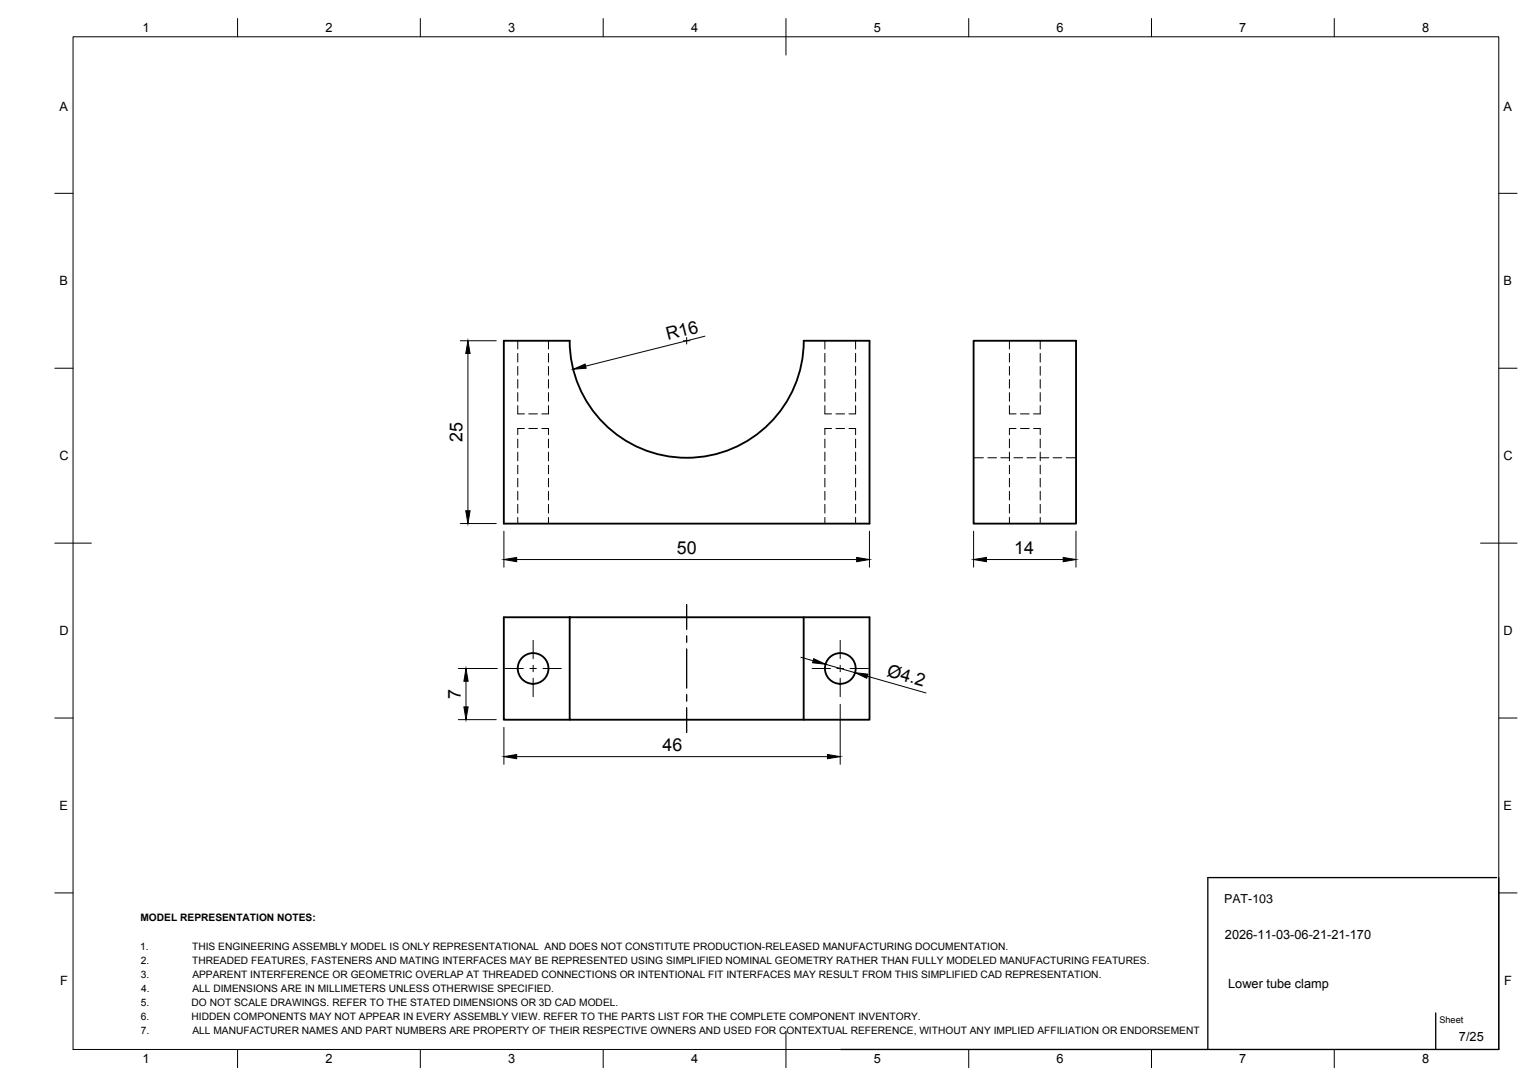
ISO-10303-21;
HEADER;
/* Generated by software containing ST-Developer
 * from STEP Tools, Inc. (www.steptools.com) 
 */

FILE_DESCRIPTION(
/* description */ ('Telescoping shaft support with lock collar'),
/* implementation_level */ '2;1');

FILE_NAME(
/* name */ 'Lower tube clamp.step',
/* time_stamp */ '2026-10-27T10:48:51-07:00',
/* author */ (''),
/* organization */ (''),
/* preprocessor_version */ 'ST-DEVELOPER v20.2',
/* originating_system */ 'Autodesk Translation Framework v15.17.0.0',
/* authorisation */ '');

FILE_SCHEMA (('AUTOMOTIVE_DESIGN { 1 0 10303 214 3 1 1 }'));
ENDSEC;

DATA;
#10=MECHANICAL_DESIGN_GEOMETRIC_PRESENTATION_REPRESENTATION('',(#243),#7349);
#203=SHAPE_REPRESENTATION_RELATIONSHIP('SRR','None',#7445,#223);
#223=ADVANCED_BREP_SHAPE_REPRESENTATION('',(#263),#7329);
#243=STYLED_ITEM('',(#7613),#263);
#263=MANIFOLD_SOLID_BREP('Body1',#3966);
#297=FACE_BOUND('',#780,.T.);
#298=FACE_BOUND('',#785,.T.);
#299=FACE_BOUND('',#787,.T.);
#300=FACE_BOUND('',#788,.T.);
#375=PLANE('',#4297);
#376=PLANE('',#4301);
#377=PLANE('',#4305);
#378=PLANE('',#4309);
#379=PLANE('',#4313);
#380=PLANE('',#4314);
#381=PLANE('',#4315);
#382=PLANE('',#4316);
#383=PLANE('',#4317);
#384=PLANE('',#4318);
#385=PLANE('',#4319);
#525=FACE_OUTER_BOUND('',#769,.T.);
#526=FACE_OUTER_BOUND('',#770,.T.);
#527=FACE_OUTER_BOUND('',#771,.T.);
#528=FACE_OUTER_BOUND('',#772,.T.);
#529=FACE_OUTER_BOUND('',#773,.T.);
#530=FACE_OUTER_BOUND('',#774,.T.);
#531=FACE_OUTER_BOUND('',#775,.T.);
#532=FACE_OUTER_BOUND('',#776,.T.);
#533=FACE_OUTER_BOUND('',#777,.T.);
#534=FACE_OUTER_BOUND('',#778,.T.);
#535=FACE_OUTER_BOUND('',#779,.T.);
#536=FACE_OUTER_BOUND('',#781,.T.);
#537=FACE_OUTER_BOUND('',#782,.T.);
#538=FACE_OUTER_BOUND('',#783,.T.);
#539=FACE_OUTER_BOUND('',#784,.T.);
#540=FACE_OUTER_BOUND('',#786,.T.);
#769=EDGE_LOOP('',(#2822,#2823,#2824,#2825));
#770=EDGE_LOOP('',(#2826));
#771=EDGE_LOOP('',(#2827,#2828,#2829,#2830));
#772=EDGE_LOOP('',(#2831));
#773=EDGE_LOOP('',(#2832,#2833,#2834,#2835));
#774=EDGE_LOOP('',(#2836));
#775=EDGE_LOOP('',(#2837,#2838,#2839,#2840));
#776=EDGE_LOOP('',(#2841));
#777=EDGE_LOOP('',(#2842,#2843,#2844,#2845));
#778=EDGE_LOOP('',(#2846,#2847,#2848,#2849,#2850,#2851));
#779=EDGE_LOOP('',(#2852,#2853,#2854,#2855));
#780=EDGE_LOOP('',(#2856));
#781=EDGE_LOOP('',(#2857,#2858,#2859,#2860));
#782=EDGE_LOOP('',(#2861,#2862,#2863,#2864));
#783=EDGE_LOOP('',(#2865,#2866,#2867,#2868,#2869,#2870));
#784=EDGE_LOOP('',(#2871,#2872,#2873,#2874));
#785=EDGE_LOOP('',(#2875));
#786=EDGE_LOOP('',(#2876,#2877,#2878,#2879));
#787=EDGE_LOOP('',(#2880));
#788=EDGE_LOOP('',(#2881));
#1065=LINE('',#6176,#1345);
#1066=LINE('',#6183,#1346);
#1067=LINE('',#6190,#1347);
#1068=LINE('',#6197,#1348);
#1069=LINE('',#6205,#1349);
#1070=LINE('',#6208,#1350);
#1071=LINE('',#6211,#1351);
#1072=LINE('',#6213,#1352);
#1073=LINE('',#6215,#1353);
#1074=LINE('',#6217,#1354);
#1075=LINE('',#6218,#1355);
#1076=LINE('',#6221,#1356);
#1077=LINE('',#6222,#1357);
#1078=LINE('',#6225,#1358);
#1079=LINE('',#6227,#1359);
#1080=LINE('',#6228,#1360);
#1081=LINE('',#6231,#1361);
#1082=LINE('',#6232,#1362);
#1083=LINE('',#6234,#1363);
#1084=LINE('',#6235,#1364);
#1345=VECTOR('',#4923,0.21);
#1346=VECTOR('',#4932,0.21);
#1347=VECTOR('',#4941,0.21);
#1348=VECTOR('',#4950,0.21);
#1349=VECTOR('',#4959,1.);
#1350=VECTOR('',#4962,1.);
#1351=VECTOR('',#4965,1.);
#1352=VECTOR('',#4966,1.);
#1353=VECTOR('',#4967,1.);
#1354=VECTOR('',#4968,1.);
#1355=VECTOR('',#4969,1.);
#1356=VECTOR('',#4972,1.);
#1357=VECTOR('',#4973,1.);
#1358=VECTOR('',#4976,1.);
#1359=VECTOR('',#4977,1.);
#1360=VECTOR('',#4978,1.);
#1361=VECTOR('',#4981,1.);
#1362=VECTOR('',#4982,1.);
#1363=VECTOR('',#4985,1.);
#1364=VECTOR('',#4986,1.);
#1639=CIRCLE('',#4295,0.21);
#1640=CIRCLE('',#4296,0.21);
#1641=CIRCLE('',#4299,0.21);
#1642=CIRCLE('',#4300,0.21);
#1643=CIRCLE('',#4303,0.21);
#1644=CIRCLE('',#4304,0.21);
#1645=CIRCLE('',#4307,0.21);
#1646=CIRCLE('',#4308,0.21);
#1647=CIRCLE('',#4311,1.6);
#1648=CIRCLE('',#4312,1.6);
#1858=VERTEX_POINT('',#6173);
#1859=VERTEX_POINT('',#6175);
#1860=VERTEX_POINT('',#6180);
#1861=VERTEX_POINT('',#6182);
#1862=VERTEX_POINT('',#6187);
#1863=VERTEX_POINT('',#6189);
#1864=VERTEX_POINT('',#6194);
#1865=VERTEX_POINT('',#6196);
#1866=VERTEX_POINT('',#6201);
#1867=VERTEX_POINT('',#6202);
#1868=VERTEX_POINT('',#6204);
#1869=VERTEX_POINT('',#6206);
#1870=VERTEX_POINT('',#6210);
#1871=VERTEX_POINT('',#6212);
#1872=VERTEX_POINT('',#6214);
#1873=VERTEX_POINT('',#6216);
#1874=VERTEX_POINT('',#6220);
#1875=VERTEX_POINT('',#6224);
#1876=VERTEX_POINT('',#6226);
#1877=VERTEX_POINT('',#6230);
#2223=EDGE_CURVE('',#1858,#1858,#1639,.T.);
#2224=EDGE_CURVE('',#1858,#1859,#1065,.T.);
#2225=EDGE_CURVE('',#1859,#1859,#1640,.T.);
#2226=EDGE_CURVE('',#1860,#1860,#1641,.T.);
#2227=EDGE_CURVE('',#1860,#1861,#1066,.T.);
#2228=EDGE_CURVE('',#1861,#1861,#1642,.T.);
#2229=EDGE_CURVE('',#1862,#1862,#1643,.T.);
#2230=EDGE_CURVE('',#1862,#1863,#1067,.T.);
#2231=EDGE_CURVE('',#1863,#1863,#1644,.T.);
#2232=EDGE_CURVE('',#1864,#1864,#1645,.T.);
#2233=EDGE_CURVE('',#1864,#1865,#1068,.T.);
#2234=EDGE_CURVE('',#1865,#1865,#1646,.T.);
#2235=EDGE_CURVE('',#1866,#1867,#1647,.T.);
#2236=EDGE_CURVE('',#1868,#1866,#1069,.T.);
#2237=EDGE_CURVE('',#1869,#1868,#1648,.T.);
#2238=EDGE_CURVE('',#1867,#1869,#1070,.T.);
#2239=EDGE_CURVE('',#1870,#1868,#1071,.T.);
#2240=EDGE_CURVE('',#1871,#1870,#1072,.T.);
#2241=EDGE_CURVE('',#1871,#1872,#1073,.T.);
#2242=EDGE_CURVE('',#1872,#1873,#1074,.T.);
#2243=EDGE_CURVE('',#1869,#1873,#1075,.T.);
#2244=EDGE_CURVE('',#1866,#1874,#1076,.T.);
#2245=EDGE_CURVE('',#1874,#1870,#1077,.T.);
#2246=EDGE_CURVE('',#1872,#1875,#1078,.T.);
#2247=EDGE_CURVE('',#1875,#1876,#1079,.T.);
#2248=EDGE_CURVE('',#1873,#1876,#1080,.T.);
#2249=EDGE_CURVE('',#1877,#1871,#1081,.T.);
#2250=EDGE_CURVE('',#1877,#1874,#1082,.T.);
#2251=EDGE_CURVE('',#1876,#1867,#1083,.T.);
#2252=EDGE_CURVE('',#1875,#1877,#1084,.T.);
#2822=ORIENTED_EDGE('',*,*,#2223,.F.);
#2823=ORIENTED_EDGE('',*,*,#2224,.T.);
#2824=ORIENTED_EDGE('',*,*,#2225,.F.);
#2825=ORIENTED_EDGE('',*,*,#2224,.F.);
#2826=ORIENTED_EDGE('',*,*,#2223,.T.);
#2827=ORIENTED_EDGE('',*,*,#2226,.F.);
#2828=ORIENTED_EDGE('',*,*,#2227,.T.);
#2829=ORIENTED_EDGE('',*,*,#2228,.F.);
#2830=ORIENTED_EDGE('',*,*,#2227,.F.);
#2831=ORIENTED_EDGE('',*,*,#2226,.T.);
#2832=ORIENTED_EDGE('',*,*,#2229,.F.);
#2833=ORIENTED_EDGE('',*,*,#2230,.T.);
#2834=ORIENTED_EDGE('',*,*,#2231,.T.);
#2835=ORIENTED_EDGE('',*,*,#2230,.F.);
#2836=ORIENTED_EDGE('',*,*,#2231,.F.);
#2837=ORIENTED_EDGE('',*,*,#2232,.F.);
#2838=ORIENTED_EDGE('',*,*,#2233,.T.);
#2839=ORIENTED_EDGE('',*,*,#2234,.T.);
#2840=ORIENTED_EDGE('',*,*,#2233,.F.);
#2841=ORIENTED_EDGE('',*,*,#2234,.F.);
#2842=ORIENTED_EDGE('',*,*,#2235,.F.);
#2843=ORIENTED_EDGE('',*,*,#2236,.F.);
#2844=ORIENTED_EDGE('',*,*,#2237,.F.);
#2845=ORIENTED_EDGE('',*,*,#2238,.F.);
#2846=ORIENTED_EDGE('',*,*,#2237,.T.);
#2847=ORIENTED_EDGE('',*,*,#2239,.F.);
#2848=ORIENTED_EDGE('',*,*,#2240,.F.);
#2849=ORIENTED_EDGE('',*,*,#2241,.T.);
#2850=ORIENTED_EDGE('',*,*,#2242,.T.);
#2851=ORIENTED_EDGE('',*,*,#2243,.F.);
#2852=ORIENTED_EDGE('',*,*,#2236,.T.);
#2853=ORIENTED_EDGE('',*,*,#2244,.T.);
#2854=ORIENTED_EDGE('',*,*,#2245,.T.);
#2855=ORIENTED_EDGE('',*,*,#2239,.T.);
#2856=ORIENTED_EDGE('',*,*,#2225,.T.);
#2857=ORIENTED_EDGE('',*,*,#2246,.T.);
#2858=ORIENTED_EDGE('',*,*,#2247,.T.);
#2859=ORIENTED_EDGE('',*,*,#2248,.F.);
#2860=ORIENTED_EDGE('',*,*,#2242,.F.);
#2861=ORIENTED_EDGE('',*,*,#2249,.T.);
#2862=ORIENTED_EDGE('',*,*,#2240,.T.);
#2863=ORIENTED_EDGE('',*,*,#2245,.F.);
#2864=ORIENTED_EDGE('',*,*,#2250,.F.);
#2865=ORIENTED_EDGE('',*,*,#2235,.T.);
#2866=ORIENTED_EDGE('',*,*,#2251,.F.);
#2867=ORIENTED_EDGE('',*,*,#2247,.F.);
#2868=ORIENTED_EDGE('',*,*,#2252,.T.);
#2869=ORIENTED_EDGE('',*,*,#2250,.T.);
#2870=ORIENTED_EDGE('',*,*,#2244,.F.);
#2871=ORIENTED_EDGE('',*,*,#2238,.T.);
#2872=ORIENTED_EDGE('',*,*,#2243,.T.);
#2873=ORIENTED_EDGE('',*,*,#2248,.T.);
#2874=ORIENTED_EDGE('',*,*,#2251,.T.);
#2875=ORIENTED_EDGE('',*,*,#2228,.T.);
#2876=ORIENTED_EDGE('',*,*,#2252,.F.);
#2877=ORIENTED_EDGE('',*,*,#2246,.F.);
#2878=ORIENTED_EDGE('',*,*,#2241,.F.);
#2879=ORIENTED_EDGE('',*,*,#2249,.F.);
#2880=ORIENTED_EDGE('',*,*,#2229,.T.);
#2881=ORIENTED_EDGE('',*,*,#2232,.T.);
#3674=CYLINDRICAL_SURFACE('',#4294,0.21);
#3675=CYLINDRICAL_SURFACE('',#4298,0.21);
#3676=CYLINDRICAL_SURFACE('',#4302,0.21);
#3677=CYLINDRICAL_SURFACE('',#4306,0.21);
#3678=CYLINDRICAL_SURFACE('',#4310,1.6);
#3768=ADVANCED_FACE('',(#525),#3674,.F.);
#3769=ADVANCED_FACE('',(#526),#375,.T.);
#3770=ADVANCED_FACE('',(#527),#3675,.F.);
#3771=ADVANCED_FACE('',(#528),#376,.T.);
#3772=ADVANCED_FACE('',(#529),#3676,.F.);
#3773=ADVANCED_FACE('',(#530),#377,.F.);
#3774=ADVANCED_FACE('',(#531),#3677,.F.);
#3775=ADVANCED_FACE('',(#532),#378,.F.);
#3776=ADVANCED_FACE('',(#533),#3678,.F.);
#3777=ADVANCED_FACE('',(#534),#379,.T.);
#3778=ADVANCED_FACE('',(#535,#297),#380,.T.);
#3779=ADVANCED_FACE('',(#536),#381,.T.);
#3780=ADVANCED_FACE('',(#537),#382,.T.);
#3781=ADVANCED_FACE('',(#538),#383,.T.);
#3782=ADVANCED_FACE('',(#539,#298),#384,.T.);
#3783=ADVANCED_FACE('',(#540,#299,#300),#385,.F.);
#3966=CLOSED_SHELL('',(#3768,#3769,#3770,#3771,#3772,#3773,#3774,#3775,
#3776,#3777,#3778,#3779,#3780,#3781,#3782,#3783));
#4293=AXIS2_PLACEMENT_3D('',#6171,#4917,#4918);
#4294=AXIS2_PLACEMENT_3D('',#6172,#4919,#4920);
#4295=AXIS2_PLACEMENT_3D('',#6174,#4921,#4922);
#4296=AXIS2_PLACEMENT_3D('',#6177,#4924,#4925);
#4297=AXIS2_PLACEMENT_3D('',#6178,#4926,#4927);
#4298=AXIS2_PLACEMENT_3D('',#6179,#4928,#4929);
#4299=AXIS2_PLACEMENT_3D('',#6181,#4930,#4931);
#4300=AXIS2_PLACEMENT_3D('',#6184,#4933,#4934);
#4301=AXIS2_PLACEMENT_3D('',#6185,#4935,#4936);
#4302=AXIS2_PLACEMENT_3D('',#6186,#4937,#4938);
#4303=AXIS2_PLACEMENT_3D('',#6188,#4939,#4940);
#4304=AXIS2_PLACEMENT_3D('',#6191,#4942,#4943);
#4305=AXIS2_PLACEMENT_3D('',#6192,#4944,#4945);
#4306=AXIS2_PLACEMENT_3D('',#6193,#4946,#4947);
#4307=AXIS2_PLACEMENT_3D('',#6195,#4948,#4949);
#4308=AXIS2_PLACEMENT_3D('',#6198,#4951,#4952);
#4309=AXIS2_PLACEMENT_3D('',#6199,#4953,#4954);
#4310=AXIS2_PLACEMENT_3D('',#6200,#4955,#4956);
#4311=AXIS2_PLACEMENT_3D('',#6203,#4957,#4958);
#4312=AXIS2_PLACEMENT_3D('',#6207,#4960,#4961);
#4313=AXIS2_PLACEMENT_3D('',#6209,#4963,#4964);
#4314=AXIS2_PLACEMENT_3D('',#6219,#4970,#4971);
#4315=AXIS2_PLACEMENT_3D('',#6223,#4974,#4975);
#4316=AXIS2_PLACEMENT_3D('',#6229,#4979,#4980);
#4317=AXIS2_PLACEMENT_3D('',#6233,#4983,#4984);
#4318=AXIS2_PLACEMENT_3D('',#6236,#4987,#4988);
#4319=AXIS2_PLACEMENT_3D('',#6237,#4989,#4990);
#4917=DIRECTION('axis',(0.,0.,1.));
#4918=DIRECTION('refdir',(1.,0.,0.));
#4919=DIRECTION('center_axis',(0.,0.,1.));
#4920=DIRECTION('ref_axis',(1.,0.,0.));
#4921=DIRECTION('center_axis',(0.,0.,1.));
#4922=DIRECTION('ref_axis',(1.,0.,0.));
#4923=DIRECTION('',(0.,0.,1.));
#4924=DIRECTION('center_axis',(0.,0.,-1.));
#4925=DIRECTION('ref_axis',(1.,0.,0.));
#4926=DIRECTION('center_axis',(0.,0.,1.));
#4927=DIRECTION('ref_axis',(1.,0.,0.));
#4928=DIRECTION('center_axis',(0.,0.,1.));
#4929=DIRECTION('ref_axis',(1.,0.,0.));
#4930=DIRECTION('center_axis',(0.,0.,1.));
#4931=DIRECTION('ref_axis',(1.,0.,0.));
#4932=DIRECTION('',(0.,0.,1.));
#4933=DIRECTION('center_axis',(0.,0.,-1.));
#4934=DIRECTION('ref_axis',(1.,0.,0.));
#4935=DIRECTION('center_axis',(0.,0.,1.));
#4936=DIRECTION('ref_axis',(1.,0.,0.));
#4937=DIRECTION('center_axis',(0.,0.,1.));
#4938=DIRECTION('ref_axis',(1.,0.,0.));
#4939=DIRECTION('center_axis',(0.,0.,1.));
#4940=DIRECTION('ref_axis',(1.,0.,0.));
#4941=DIRECTION('',(0.,0.,1.));
#4942=DIRECTION('center_axis',(0.,0.,1.));
#4943=DIRECTION('ref_axis',(1.,0.,0.));
#4944=DIRECTION('center_axis',(0.,0.,1.));
#4945=DIRECTION('ref_axis',(1.,0.,0.));
#4946=DIRECTION('center_axis',(0.,0.,1.));
#4947=DIRECTION('ref_axis',(1.,0.,0.));
#4948=DIRECTION('center_axis',(0.,0.,1.));
#4949=DIRECTION('ref_axis',(1.,0.,0.));
#4950=DIRECTION('',(0.,0.,1.));
#4951=DIRECTION('center_axis',(0.,0.,1.));
#4952=DIRECTION('ref_axis',(1.,0.,0.));
#4953=DIRECTION('center_axis',(0.,0.,1.));
#4954=DIRECTION('ref_axis',(1.,0.,0.));
#4955=DIRECTION('center_axis',(1.,0.,0.));
#4956=DIRECTION('ref_axis',(0.,0.,-1.));
#4957=DIRECTION('center_axis',(1.,0.,0.));
#4958=DIRECTION('ref_axis',(0.,0.,-1.));
#4959=DIRECTION('',(-1.,0.,0.));
#4960=DIRECTION('center_axis',(-1.,0.,0.));
#4961=DIRECTION('ref_axis',(0.,0.,-1.));
#4962=DIRECTION('',(1.,0.,0.));
#4963=DIRECTION('center_axis',(1.,0.,0.));
#4964=DIRECTION('ref_axis',(0.,1.,0.));
#4965=DIRECTION('',(0.,1.,0.));
#4966=DIRECTION('',(0.,0.,1.));
#4967=DIRECTION('',(0.,1.,0.));
#4968=DIRECTION('',(0.,0.,1.));
#4969=DIRECTION('',(0.,1.,0.));
#4970=DIRECTION('center_axis',(0.,0.,1.));
#4971=DIRECTION('ref_axis',(1.,0.,0.));
#4972=DIRECTION('',(0.,-1.,0.));
#4973=DIRECTION('',(1.,0.,0.));
#4974=DIRECTION('center_axis',(0.,1.,0.));
#4975=DIRECTION('ref_axis',(-1.,0.,0.));
#4976=DIRECTION('',(-1.,0.,0.));
#4977=DIRECTION('',(0.,0.,1.));
#4978=DIRECTION('',(-1.,0.,0.));
#4979=DIRECTION('center_axis',(0.,-1.,0.));
#4980=DIRECTION('ref_axis',(1.,0.,0.));
#4981=DIRECTION('',(1.,0.,0.));
#4982=DIRECTION('',(0.,0.,1.));
#4983=DIRECTION('center_axis',(-1.,0.,0.));
#4984=DIRECTION('ref_axis',(0.,-1.,0.));
#4985=DIRECTION('',(0.,-1.,0.));
#4986=DIRECTION('',(0.,-1.,0.));
#4987=DIRECTION('center_axis',(0.,0.,1.));
#4988=DIRECTION('ref_axis',(1.,0.,0.));
#4989=DIRECTION('center_axis',(0.,0.,1.));
#4990=DIRECTION('ref_axis',(1.,0.,0.));
#6171=CARTESIAN_POINT('',(0.,0.,0.));
#6172=CARTESIAN_POINT('Origin',(2.2,-2.1,2.5));
#6173=CARTESIAN_POINT('',(1.99,-2.1,2.5));
#6174=CARTESIAN_POINT('Origin',(2.2,-2.1,2.5));
#6175=CARTESIAN_POINT('',(1.99,-2.1,3.5));
#6176=CARTESIAN_POINT('',(1.99,-2.1,2.5));
#6177=CARTESIAN_POINT('Origin',(2.2,-2.1,3.5));
#6178=CARTESIAN_POINT('Origin',(2.2,-2.1,2.5));
#6179=CARTESIAN_POINT('Origin',(2.2,2.1,2.5));
#6180=CARTESIAN_POINT('',(1.99,2.1,2.5));
#6181=CARTESIAN_POINT('Origin',(2.2,2.1,2.5));
#6182=CARTESIAN_POINT('',(1.99,2.1,3.5));
#6183=CARTESIAN_POINT('',(1.99,2.1,2.5));
#6184=CARTESIAN_POINT('Origin',(2.2,2.1,3.5));
#6185=CARTESIAN_POINT('Origin',(2.2,2.1,2.5));
#6186=CARTESIAN_POINT('Origin',(2.2,-2.1,0.9));
#6187=CARTESIAN_POINT('',(1.99,-2.1,1.));
#6188=CARTESIAN_POINT('Origin',(2.2,-2.1,1.));
#6189=CARTESIAN_POINT('',(1.99,-2.1,2.3));
#6190=CARTESIAN_POINT('',(1.99,-2.1,0.9));
#6191=CARTESIAN_POINT('Origin',(2.2,-2.1,2.3));
#6192=CARTESIAN_POINT('Origin',(2.2,-2.1,2.3));
#6193=CARTESIAN_POINT('Origin',(2.2,2.1,0.9));
#6194=CARTESIAN_POINT('',(1.99,2.1,1.));
#6195=CARTESIAN_POINT('Origin',(2.2,2.1,1.));
#6196=CARTESIAN_POINT('',(1.99,2.1,2.3));
#6197=CARTESIAN_POINT('',(1.99,2.1,0.9));
#6198=CARTESIAN_POINT('Origin',(2.2,2.1,2.3));
#6199=CARTESIAN_POINT('Origin',(2.2,2.1,2.3));
#6200=CARTESIAN_POINT('Origin',(1.4,0.,3.5));
#6201=CARTESIAN_POINT('',(1.5,-1.6,3.5));
#6202=CARTESIAN_POINT('',(1.5,1.6,3.5));
#6203=CARTESIAN_POINT('Origin',(1.5,0.,3.5));
#6204=CARTESIAN_POINT('',(2.9,-1.6,3.5));
#6205=CARTESIAN_POINT('',(1.4,-1.6,3.5));
#6206=CARTESIAN_POINT('',(2.9,1.6,3.5));
#6207=CARTESIAN_POINT('Origin',(2.9,0.,3.5));
#6208=CARTESIAN_POINT('',(1.4,1.6,3.5));
#6209=CARTESIAN_POINT('Origin',(2.9,-2.5,1.));
#6210=CARTESIAN_POINT('',(2.9,-2.5,3.5));
#6211=CARTESIAN_POINT('',(2.9,-2.5,3.5));
#6212=CARTESIAN_POINT('',(2.9,-2.5,1.));
#6213=CARTESIAN_POINT('',(2.9,-2.5,1.));
#6214=CARTESIAN_POINT('',(2.9,2.5,1.));
#6215=CARTESIAN_POINT('',(2.9,-2.5,1.));
#6216=CARTESIAN_POINT('',(2.9,2.5,3.5));
#6217=CARTESIAN_POINT('',(2.9,2.5,1.));
#6218=CARTESIAN_POINT('',(2.9,-2.5,3.5));
#6219=CARTESIAN_POINT('Origin',(2.2,0.,3.5));
#6220=CARTESIAN_POINT('',(1.5,-2.5,3.5));
#6221=CARTESIAN_POINT('',(1.5,2.5,3.5));
#6222=CARTESIAN_POINT('',(1.5,-2.5,3.5));
#6223=CARTESIAN_POINT('Origin',(2.9,2.5,1.));
#6224=CARTESIAN_POINT('',(1.5,2.5,1.));
#6225=CARTESIAN_POINT('',(2.9,2.5,1.));
#6226=CARTESIAN_POINT('',(1.5,2.5,3.5));
#6227=CARTESIAN_POINT('',(1.5,2.5,1.));
#6228=CARTESIAN_POINT('',(2.9,2.5,3.5));
#6229=CARTESIAN_POINT('Origin',(1.5,-2.5,1.));
#6230=CARTESIAN_POINT('',(1.5,-2.5,1.));
#6231=CARTESIAN_POINT('',(1.5,-2.5,1.));
#6232=CARTESIAN_POINT('',(1.5,-2.5,1.));
#6233=CARTESIAN_POINT('Origin',(1.5,2.5,1.));
#6234=CARTESIAN_POINT('',(1.5,2.5,3.5));
#6235=CARTESIAN_POINT('',(1.5,2.5,1.));
#6236=CARTESIAN_POINT('Origin',(2.2,0.,3.5));
#6237=CARTESIAN_POINT('Origin',(2.2,0.,1.));
#7304=UNCERTAINTY_MEASURE_WITH_UNIT(LENGTH_MEASURE(0.001),#7350,
'DISTANCE_ACCURACY_VALUE',
'Maximum model space distance between geometric entities at asserted c
onnectivities');
#7324=UNCERTAINTY_MEASURE_WITH_UNIT(LENGTH_MEASURE(0.001),#7350,
'DISTANCE_ACCURACY_VALUE',
'Maximum model space distance between geometric entities at asserted c
onnectivities');
#7329=(
GEOMETRIC_REPRESENTATION_CONTEXT(3)
GLOBAL_UNCERTAINTY_ASSIGNED_CONTEXT((#7304))
GLOBAL_UNIT_ASSIGNED_CONTEXT((#7350,#7352,#7353))
REPRESENTATION_CONTEXT('','3D')
);
#7349=(
GEOMETRIC_REPRESENTATION_CONTEXT(3)
GLOBAL_UNCERTAINTY_ASSIGNED_CONTEXT((#7324))
GLOBAL_UNIT_ASSIGNED_CONTEXT((#7350,#7352,#7353))
REPRESENTATION_CONTEXT('','3D')
);
#7350=(
LENGTH_UNIT()
NAMED_UNIT(*)
SI_UNIT(.CENTI.,.METRE.)
);
#7352=(
NAMED_UNIT(*)
PLANE_ANGLE_UNIT()
SI_UNIT($,.RADIAN.)
);
#7353=(
NAMED_UNIT(*)
SI_UNIT($,.STERADIAN.)
SOLID_ANGLE_UNIT()
);
#7358=SHAPE_DEFINITION_REPRESENTATION(#7382,#7445);
#7382=PRODUCT_DEFINITION_SHAPE('',$,#7470);
#7445=SHAPE_REPRESENTATION('',(#4293),#7329);
#7465=PRODUCT_DEFINITION_CONTEXT('part definition',#7539,'design');
#7470=PRODUCT_DEFINITION('Lower tube clamp','Lower tube clamp',#7494,#7465);
#7494=PRODUCT_DEFINITION_FORMATION('',$,#7545);
#7539=APPLICATION_CONTEXT(
'Core Data for Automotive Mechanical Design Process');
#7540=PRODUCT_CONTEXT('part definition',#7539,'mechanical');
#7545=PRODUCT('Lower tube clamp','Lower tube clamp','Lower tube clamp',
(#7540));
#7607=COLOUR_RGB('Light Blue',0.38,0.62,0.78);
#7608=FILL_AREA_STYLE_COLOUR('',#7607);
#7609=FILL_AREA_STYLE('',(#7608));
#7610=SURFACE_STYLE_FILL_AREA(#7609);
#7611=SURFACE_SIDE_STYLE('',(#7610));
#7612=SURFACE_STYLE_USAGE(.BOTH.,#7611);
#7613=PRESENTATION_STYLE_ASSIGNMENT((#7612));
ENDSEC;
END-ISO-10303-21;
